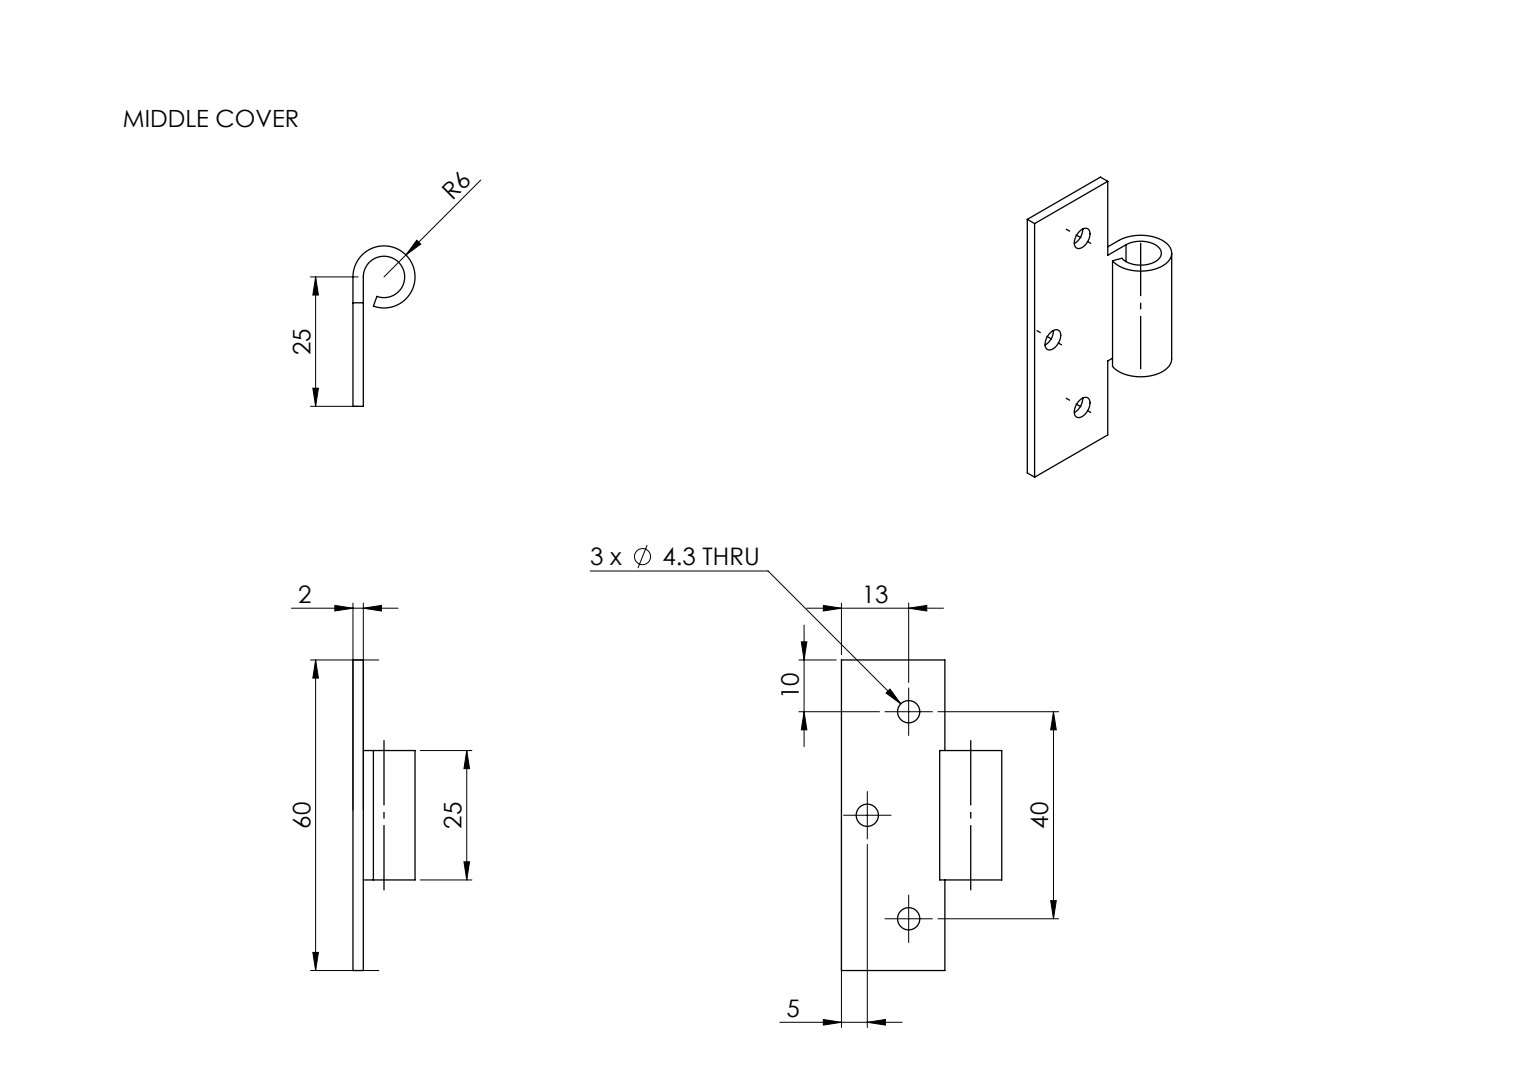
ISO-10303-21;
HEADER;
FILE_DESCRIPTION (('STEP AP214'),
    '1' );
FILE_NAME ('middle cover.step',
    '2026-10-03T20:08:58',
    ( '' ),
    ( '' ),
    'SwSTEP 2.0',
    'SolidWorks 2026',
    '' );
FILE_SCHEMA (( 'AUTOMOTIVE_DESIGN' ));
ENDSEC;

DATA;
#53=ORIENTED_EDGE ( 'NONE', *, *, #9830, .F. ) ;
#58=ORIENTED_EDGE ( 'NONE', *, *, #11138, .F. ) ;
#71=SHAPE_REPRESENTATION ( 'middle cover', ( #12422 ), #3113 ) ;
#124=VECTOR ( 'NONE', #5391, 1000.000000000000000 ) ;
#153=CYLINDRICAL_SURFACE ( 'NONE', #2365, 2.149999999999999023 ) ;
#185=CARTESIAN_POINT ( 'NONE',  ( 15.00000000000003375, -12.49999999999999645, 3.994800001834461867E-31 ) ) ;
#198=DIRECTION ( 'NONE',  ( 1.000000000000000000, 1.849040895279789448E-31, -6.938893903907224680E-17 ) ) ;
#203=CARTESIAN_POINT ( 'NONE',  ( 15.00000000000003375, 30.00000000000001776, -9.742497179615118866E-31 ) ) ;
#207=ORIENTED_EDGE ( 'NONE', *, *, #11487, .T. ) ;
#225=CYLINDRICAL_SURFACE ( 'NONE', #8627, 4.000000000000008882 ) ;
#265=AXIS2_PLACEMENT_3D ( 'NONE', #2707, #625, #8413 ) ;
#298=ORIENTED_EDGE ( 'NONE', *, *, #6646, .F. ) ;
#306=EDGE_CURVE ( 'NONE', #7136, #2489, #7613, .T. ) ;
#307=FACE_OUTER_BOUND ( 'NONE', #3872, .T. ) ;
#324=FACE_BOUND ( 'NONE', #7382, .T. ) ;
#328=DIRECTION ( 'NONE',  ( 1.000000000000000000, 1.849040895279789448E-31, -6.938893903907224680E-17 ) ) ;
#331=CARTESIAN_POINT ( 'NONE',  ( 15.00000000000003375, 12.50000000000000000, -4.062508476441825628E-31 ) ) ;
#347=FACE_OUTER_BOUND ( 'NONE', #4727, .T. ) ;
#349=VERTEX_POINT ( 'NONE', #907 ) ;
#361=LINE ( 'NONE', #555, #3321 ) ;
#392=CARTESIAN_POINT ( 'NONE',  ( 11.00000000000003730, -19.99999999999999645, 12.00000000000003553 ) ) ;
#398=VECTOR ( 'NONE', #6706, 1000.000000000000000 ) ;
#415=ADVANCED_FACE ( 'NONE', ( #12584 ), #4715, .F. ) ;
#499=VERTEX_POINT ( 'NONE', #4254 ) ;
#502=VECTOR ( 'NONE', #1677, 1000.000000000000000 ) ;
#508=LINE ( 'NONE', #572, #8236 ) ;
#527=EDGE_CURVE ( 'NONE', #837, #2437, #10330, .T. ) ;
#534=CARTESIAN_POINT ( 'NONE',  ( 11.00000000000003020, 30.00000000000000000, 25.00000000000007105 ) ) ;
#539=ADVANCED_FACE ( 'NONE', ( #7031 ), #4318, .F. ) ;
#550=AXIS2_PLACEMENT_3D ( 'NONE', #4921, #8783, #1827 ) ;
#555=CARTESIAN_POINT ( 'NONE',  ( 11.00000000000003020, -30.00000000000000000, 25.00000000000007105 ) ) ;
#572=CARTESIAN_POINT ( 'NONE',  ( 11.00000000000003020, 30.00000000000000000, 5.000000000000004441 ) ) ;
#576=EDGE_CURVE ( 'NONE', #499, #3763, #3136, .T. ) ;
#604=ORIENTED_EDGE ( 'NONE', *, *, #7620, .T. ) ;
#619=PLANE ( 'NONE',  #7619 ) ;
#625=DIRECTION ( 'NONE',  ( -1.848892746611746419E-31, -1.000000000000000000, 3.250006781153460502E-32 ) ) ;
#673=CARTESIAN_POINT ( 'NONE',  ( 11.00000000000003020, 30.00000000000000000, 25.00000000000007105 ) ) ;
#705=CARTESIAN_POINT ( 'NONE',  ( 13.63191942669736889, 12.50000000000000000, 3.758770483143645702 ) ) ;
#730=ORIENTED_EDGE ( 'NONE', *, *, #7700, .F. ) ;
#737=DIRECTION ( 'NONE',  ( -1.848892746611746419E-31, -1.000000000000000000, 3.250006781153460502E-32 ) ) ;
#772=EDGE_CURVE ( 'NONE', #5440, #1077, #5854, .T. ) ;
#773=ORIENTED_EDGE ( 'NONE', *, *, #7954, .F. ) ;
#786=UNCERTAINTY_MEASURE_WITH_UNIT (LENGTH_MEASURE( 1.000000000000000082E-05 ), #10711, 'distance_accuracy_value', 'NONE');
#837=VERTEX_POINT ( 'NONE', #4643 ) ;
#845=AXIS2_PLACEMENT_3D ( 'NONE', #4474, #8392, #8331 ) ;
#854=EDGE_CURVE ( 'NONE', #1393, #11974, #1403, .T. ) ;
#855=AXIS2_PLACEMENT_3D ( 'NONE', #331, #8316, #6321 ) ;
#861=DIRECTION ( 'NONE',  ( 1.000000000000000000, 1.849040895279789448E-31, -6.938893903907224680E-17 ) ) ;
#870=SURFACE_STYLE_USAGE ( .BOTH. , #3124 ) ;
#873=AXIS2_PLACEMENT_3D ( 'NONE', #3980, #951, #2044 ) ;
#875=EDGE_LOOP ( 'NONE', ( #207, #9419, #4311, #1916, #9816, #12149, #7760, #7885, #10727, #12727 ) ) ;
#878=LINE ( 'NONE', #9620, #1011 ) ;
#881=DIRECTION ( 'NONE',  ( 1.000000000000000000, 1.848892746611742259E-31, -1.154721252774410375E-34 ) ) ;
#889=ORIENTED_EDGE ( 'NONE', *, *, #10751, .F. ) ;
#902=EDGE_LOOP ( 'NONE', ( #5113, #5119, #7738, #9992 ) ) ;
#907=CARTESIAN_POINT ( 'NONE',  ( 11.00000000000003375, 12.50000000000000000, -7.673627122167892852E-31 ) ) ;
#911=DIRECTION ( 'NONE',  ( 1.000000000000000000, 1.849040895279789448E-31, -6.938893903907224680E-17 ) ) ;
#912=CIRCLE ( 'NONE', #1325, 2.149999999999994138 ) ;
#937=VERTEX_POINT ( 'NONE', #12282 ) ;
#951=DIRECTION ( 'NONE',  ( -1.848892746611746419E-31, -1.000000000000000000, 3.250006781153460502E-32 ) ) ;
#996=ADVANCED_FACE ( 'NONE', ( #11245 ), #1320, .T. ) ;
#1011=VECTOR ( 'NONE', #11836, 1000.000000000000000 ) ;
#1026=ORIENTED_EDGE ( 'NONE', *, *, #306, .F. ) ;
#1038=DIRECTION ( 'NONE',  ( 0.000000000000000000, 0.000000000000000000, -1.000000000000000000 ) ) ;
#1045=VERTEX_POINT ( 'NONE', #5196 ) ;
#1077=VERTEX_POINT ( 'NONE', #673 ) ;
#1088=DIRECTION ( 'NONE',  ( 1.848892746611746419E-31, 1.000000000000000000, -3.250006781153460502E-32 ) ) ;
#1093=CARTESIAN_POINT ( 'NONE',  ( 15.00000000000003375, -12.49999999999999645, 3.994800001834461867E-31 ) ) ;
#1094=DIRECTION ( 'NONE',  ( 1.848892746611746419E-31, 1.000000000000000000, -3.250006781153460502E-32 ) ) ;
#1097=LINE ( 'NONE', #6364, #1940 ) ;
#1099=CARTESIAN_POINT ( 'NONE',  ( 11.00000000000001599, 19.99999999999999645, 12.00000000000003020 ) ) ;
#1105=EDGE_LOOP ( 'NONE', ( #9618, #8342, #10391, #889 ) ) ;
#1109=DIRECTION ( 'NONE',  ( 0.000000000000000000, 0.000000000000000000, -1.000000000000000000 ) ) ;
#1119=ORIENTED_EDGE ( 'NONE', *, *, #12538, .F. ) ;
#1126=CIRCLE ( 'NONE', #4005, 2.149999999999999023 ) ;
#1171=FILL_AREA_STYLE ('',( #3782 ) ) ;
#1172=EDGE_LOOP ( 'NONE', ( #10214, #1741, #1308, #6409 ) ) ;
#1209=ADVANCED_FACE ( 'NONE', ( #7694 ), #6611, .T. ) ;
#1223=CARTESIAN_POINT ( 'NONE',  ( 11.00000000000003020, 30.00000000000000000, 5.000000000000004441 ) ) ;
#1224=EDGE_CURVE ( 'NONE', #5846, #3671, #9624, .T. ) ;
#1232=CARTESIAN_POINT ( 'NONE',  ( 11.00000000000001599, -12.49999999999999645, 3.994800001834461867E-31 ) ) ;
#1233=( NAMED_UNIT ( * ) PLANE_ANGLE_UNIT ( ) SI_UNIT ( $, .RADIAN. ) );
#1240=CARTESIAN_POINT ( 'NONE',  ( 15.00000000000003375, 30.00000000000001776, -4.000000000000008882 ) ) ;
#1250=ORIENTED_EDGE ( 'NONE', *, *, #9318, .T. ) ;
#1294=DIRECTION ( 'NONE',  ( -1.000000000000000000, -1.848892746611742259E-31, 1.154721252774410589E-34 ) ) ;
#1308=ORIENTED_EDGE ( 'NONE', *, *, #6615, .T. ) ;
#1320=PLANE ( 'NONE',  #6991 ) ;
#1325=AXIS2_PLACEMENT_3D ( 'NONE', #1099, #911, #1880 ) ;
#1393=VERTEX_POINT ( 'NONE', #12553 ) ;
#1395=ORIENTED_EDGE ( 'NONE', *, *, #11820, .T. ) ;
#1403=CIRCLE ( 'NONE', #10259, 6.000000000000013323 ) ;
#1417=CIRCLE ( 'NONE', #8620, 4.000000000000008882 ) ;
#1421=DIRECTION ( 'NONE',  ( -1.000000000000000000, -1.848892746611742259E-31, 1.154721252774410589E-34 ) ) ;
#1463=VERTEX_POINT ( 'NONE', #7578 ) ;
#1503=CARTESIAN_POINT ( 'NONE',  ( 11.00000000000003375, -6.123233995736749519E-16, 20.00000000000003553 ) ) ;
#1524=VECTOR ( 'NONE', #6266, 1000.000000000000000 ) ;
#1531=DIRECTION ( 'NONE',  ( 1.000000000000000000, 1.849040895279789448E-31, -6.938893903907224680E-17 ) ) ;
#1542=CARTESIAN_POINT ( 'NONE',  ( 9.000000000000031974, 12.50000000000000000, 5.000000000000004441 ) ) ;
#1549=EDGE_LOOP ( 'NONE', ( #9983, #8678 ) ) ;
#1552=LINE ( 'NONE', #8256, #6421 ) ;
#1558=CARTESIAN_POINT ( 'NONE',  ( 9.000000000000031974, 12.50000000000000000, -6.000000000000017764 ) ) ;
#1567=AXIS2_PLACEMENT_3D ( 'NONE', #7065, #2171, #7130 ) ;
#1590=ORIENTED_EDGE ( 'NONE', *, *, #6258, .T. ) ;
#1604=EDGE_LOOP ( 'NONE', ( #1991, #6241, #1590, #2296, #8881, #12609, #6350, #8005 ) ) ;
#1614=CARTESIAN_POINT ( 'NONE',  ( 15.00000000000003375, 12.50000000000000000, -4.062508476441825628E-31 ) ) ;
#1677=DIRECTION ( 'NONE',  ( -1.000000000000000000, -1.848892746611742259E-31, 1.154721252774410589E-34 ) ) ;
#1706=EDGE_CURVE ( 'NONE', #1045, #7990, #1417, .T. ) ;
#1723=ORIENTED_EDGE ( 'NONE', *, *, #5620, .T. ) ;
#1724=VECTOR ( 'NONE', #2011, 1000.000000000000000 ) ;
#1741=ORIENTED_EDGE ( 'NONE', *, *, #7200, .F. ) ;
#1808=LINE ( 'NONE', #10500, #12392 ) ;
#1818=UNCERTAINTY_MEASURE_WITH_UNIT (LENGTH_MEASURE( 1.000000000000000082E-05 ), #8735, 'distance_accuracy_value', 'NONE');
#1827=DIRECTION ( 'NONE',  ( 0.000000000000000000, 4.478906847412192569E-32, -1.000000000000000000 ) ) ;
#1832=SURFACE_SIDE_STYLE ('',( #9673 ) ) ;
#1842=EDGE_CURVE ( 'NONE', #7990, #8864, #4935, .T. ) ;
#1852=CARTESIAN_POINT ( 'NONE',  ( 15.00000000000003375, -29.99999999999998224, 9.742497179615118866E-31 ) ) ;
#1855=ORIENTED_EDGE ( 'NONE', *, *, #1842, .T. ) ;
#1856=ORIENTED_EDGE ( 'NONE', *, *, #4784, .T. ) ;
#1877=AXIS2_PLACEMENT_3D ( 'NONE', #1503, #5243, #8267 ) ;
#1880=DIRECTION ( 'NONE',  ( 0.000000000000000000, 0.000000000000000000, -1.000000000000000000 ) ) ;
#1889=CARTESIAN_POINT ( 'NONE',  ( 9.000000000000031974, -6.123233995736753463E-16, 20.00000000000003553 ) ) ;
#1898=ORIENTED_EDGE ( 'NONE', *, *, #1224, .T. ) ;
#1906=ORIENTED_EDGE ( 'NONE', *, *, #11800, .T. ) ;
#1916=ORIENTED_EDGE ( 'NONE', *, *, #2991, .T. ) ;
#1918=DIRECTION ( 'NONE',  ( -1.848892746611746419E-31, -1.000000000000000000, 3.250006781153460502E-32 ) ) ;
#1937=LINE ( 'NONE', #10885, #2591 ) ;
#1940=VECTOR ( 'NONE', #5035, 1000.000000000000000 ) ;
#1943=PLANE ( 'NONE',  #2694 ) ;
#1945=ADVANCED_FACE ( 'NONE', ( #4026 ), #225, .F. ) ;
#1977=ORIENTED_EDGE ( 'NONE', *, *, #6329, .F. ) ;
#1981=EDGE_LOOP ( 'NONE', ( #7314, #3852, #8670, #1856 ) ) ;
#1991=ORIENTED_EDGE ( 'NONE', *, *, #9650, .F. ) ;
#2011=DIRECTION ( 'NONE',  ( 1.000000000000000000, 1.849040895279789448E-31, -6.938893903907224680E-17 ) ) ;
#2044=DIRECTION ( 'NONE',  ( 0.000000000000000000, 0.000000000000000000, -1.000000000000000000 ) ) ;
#2046=LINE ( 'NONE', #8931, #12274 ) ;
#2133=FACE_BOUND ( 'NONE', #2564, .T. ) ;
#2138=CARTESIAN_POINT ( 'NONE',  ( 11.00000000000003375, -19.99999999999999645, 14.15000000000003411 ) ) ;
#2156=CARTESIAN_POINT ( 'NONE',  ( 11.00000000000003375, -19.99999999999999645, 12.00000000000003553 ) ) ;
#2171=DIRECTION ( 'NONE',  ( -1.848892746611746419E-31, -1.000000000000000000, 3.250006781153460502E-32 ) ) ;
#2186=ORIENTED_EDGE ( 'NONE', *, *, #9830, .T. ) ;
#2196=FACE_OUTER_BOUND ( 'NONE', #11712, .T. ) ;
#2212=VECTOR ( 'NONE', #3263, 1000.000000000000000 ) ;
#2247=EDGE_CURVE ( 'NONE', #2437, #7453, #7218, .T. ) ;
#2257=VECTOR ( 'NONE', #11038, 1000.000000000000000 ) ;
#2279=CARTESIAN_POINT ( 'NONE',  ( 12.94787914004602847, -12.49999999999999645, 5.638155724715463890 ) ) ;
#2296=ORIENTED_EDGE ( 'NONE', *, *, #10876, .F. ) ;
#2300=DIRECTION ( 'NONE',  ( 0.000000000000000000, 0.000000000000000000, -1.000000000000000000 ) ) ;
#2315=CARTESIAN_POINT ( 'NONE',  ( 15.00000000000003375, 30.00000000000001776, -9.742497179615118866E-31 ) ) ;
#2321=CARTESIAN_POINT ( 'NONE',  ( 11.00000000000003375, -6.123233995736745575E-16, 20.00000000000003553 ) ) ;
#2341=DIRECTION ( 'NONE',  ( 0.3420201433256680468, 7.946868433027814422E-32, -0.9396926207859086499 ) ) ;
#2353=LINE ( 'NONE', #10308, #1524 ) ;
#2354=ADVANCED_FACE ( 'NONE', ( #324, #10031, #2133, #8247 ), #8180, .T. ) ;
#2365=AXIS2_PLACEMENT_3D ( 'NONE', #2156, #6804, #3958 ) ;
#2389=FACE_OUTER_BOUND ( 'NONE', #5721, .T. ) ;
#2390=EDGE_LOOP ( 'NONE', ( #9885, #4090, #6511, #7356 ) ) ;
#2418=LINE ( 'NONE', #7178, #11409 ) ;
#2429=DIRECTION ( 'NONE',  ( -0.3420201433256680468, -7.946868433027813328E-32, 0.9396926207859086499 ) ) ;
#2437=VERTEX_POINT ( 'NONE', #12311 ) ;
#2447=FACE_OUTER_BOUND ( 'NONE', #1981, .T. ) ;
#2466=EDGE_LOOP ( 'NONE', ( #12293, #4442 ) ) ;
#2468=CARTESIAN_POINT ( 'NONE',  ( 21.00000000000003197, -30.00000000000000000, 5.000000000000011546 ) ) ;
#2489=VERTEX_POINT ( 'NONE', #1542 ) ;
#2522=CIRCLE ( 'NONE', #855, 4.000000000000008882 ) ;
#2533=ORIENTED_EDGE ( 'NONE', *, *, #6615, .F. ) ;
#2564=EDGE_LOOP ( 'NONE', ( #58, #5215 ) ) ;
#2591=VECTOR ( 'NONE', #6970, 1000.000000000000000 ) ;
#2614=ORIENTED_EDGE ( 'NONE', *, *, #1706, .F. ) ;
#2636=ORIENTED_EDGE ( 'NONE', *, *, #11706, .F. ) ;
#2663=CARTESIAN_POINT ( 'NONE',  ( 9.000000000000017764, 19.99999999999999645, 14.15000000000002345 ) ) ;
#2688=ORIENTED_EDGE ( 'NONE', *, *, #7898, .T. ) ;
#2694=AXIS2_PLACEMENT_3D ( 'NONE', #203, #4132, #11745 ) ;
#2703=ORIENTED_EDGE ( 'NONE', *, *, #6258, .F. ) ;
#2707=CARTESIAN_POINT ( 'NONE',  ( 15.00000000000003375, 12.50000000000000000, -4.062508476441825628E-31 ) ) ;
#2709=PRODUCT ( 'middle cover', 'middle cover', '', ( #4085 ) ) ;
#2746=CLOSED_SHELL ( 'NONE', ( #9617, #539, #4850, #4582, #5554, #3059, #5777, #10912, #10366, #6759, #10943, #2354, #1945, #996, #1209, #7851, #11352, #7779, #415, #8563, #6522, #11560 ) ) ;
#2791=CARTESIAN_POINT ( 'NONE',  ( 15.00000000000003375, 12.50000000000000000, -4.062508476441825628E-31 ) ) ;
#2821=DIRECTION ( 'NONE',  ( 0.000000000000000000, 0.000000000000000000, -1.000000000000000000 ) ) ;
#2833=SURFACE_STYLE_FILL_AREA ( #1171 ) ;
#2835=ORIENTED_EDGE ( 'NONE', *, *, #11243, .T. ) ;
#2876=EDGE_LOOP ( 'NONE', ( #4069, #1855, #2636, #1119 ) ) ;
#2890=FILL_AREA_STYLE ('',( #12540 ) ) ;
#2896=( NAMED_UNIT ( * ) SI_UNIT ( $, .STERADIAN. ) SOLID_ANGLE_UNIT ( ) );
#2897=AXIS2_PLACEMENT_3D ( 'NONE', #9255, #5155, #7153 ) ;
#2902=DIRECTION ( 'NONE',  ( -1.848892746611746419E-31, -1.000000000000000000, 3.250006781153460502E-32 ) ) ;
#2991=EDGE_CURVE ( 'NONE', #11641, #9518, #878, .T. ) ;
#3022=DIRECTION ( 'NONE',  ( -1.848892746611746419E-31, -1.000000000000000000, 3.250006781153460502E-32 ) ) ;
#3044=VECTOR ( 'NONE', #5677, 1000.000000000000000 ) ;
#3059=ADVANCED_FACE ( 'NONE', ( #8608 ), #9684, .F. ) ;
#3072=LINE ( 'NONE', #10904, #2257 ) ;
#3076=DIRECTION ( 'NONE',  ( 1.000000000000000000, 1.849040895279789448E-31, -6.938893903907224680E-17 ) ) ;
#3081=CARTESIAN_POINT ( 'NONE',  ( 13.63191942669736889, 30.00000000000001776, 3.758770483143646146 ) ) ;
#3113=( GEOMETRIC_REPRESENTATION_CONTEXT ( 3 ) GLOBAL_UNCERTAINTY_ASSIGNED_CONTEXT ( ( #10448 ) ) GLOBAL_UNIT_ASSIGNED_CONTEXT ( ( #6131, #3843, #12064 ) ) REPRESENTATION_CONTEXT ( 'NONE', 'WORKASPACE' ) );
#3124=SURFACE_SIDE_STYLE ('',( #2833 ) ) ;
#3136=CIRCLE ( 'NONE', #4179, 4.000000000000008882 ) ;
#3156=CARTESIAN_POINT ( 'NONE',  ( 9.000000000000017764, 19.99999999999999645, 12.00000000000003020 ) ) ;
#3169=VERTEX_POINT ( 'NONE', #3337 ) ;
#3176=LINE ( 'NONE', #5517, #3290 ) ;
#3182=CARTESIAN_POINT ( 'NONE',  ( 11.00000000000003375, -6.123233995736745575E-16, 20.00000000000003553 ) ) ;
#3193=ORIENTED_EDGE ( 'NONE', *, *, #3431, .T. ) ;
#3196=AXIS2_PLACEMENT_3D ( 'NONE', #7099, #11084, #5225 ) ;
#3232=DIRECTION ( 'NONE',  ( -1.848892746611746419E-31, -1.000000000000000000, 3.250006781153460502E-32 ) ) ;
#3248=DIRECTION ( 'NONE',  ( 1.848892746611746419E-31, 1.000000000000000000, -3.250006781153460502E-32 ) ) ;
#3251=DIRECTION ( 'NONE',  ( -1.154721252774002618E-34, 1.982541115402070533E-16, 1.000000000000000000 ) ) ;
#3263=DIRECTION ( 'NONE',  ( -1.848892746611746419E-31, -1.000000000000000000, 3.250006781153460502E-32 ) ) ;
#3276=ORIENTED_EDGE ( 'NONE', *, *, #8405, .T. ) ;
#3277=CARTESIAN_POINT ( 'NONE',  ( 15.00000000000003375, 12.50000000000000000, -4.062508476441825628E-31 ) ) ;
#3290=VECTOR ( 'NONE', #8410, 1000.000000000000000 ) ;
#3291=CYLINDRICAL_SURFACE ( 'NONE', #8137, 6.000000000000013323 ) ;
#3298=DIRECTION ( 'NONE',  ( 1.848892746611746419E-31, 1.000000000000000000, -3.250006781153460502E-32 ) ) ;
#3304=CARTESIAN_POINT ( 'NONE',  ( 9.000000000000017764, -12.50000000000000178, 5.000000000000007994 ) ) ;
#3321=VECTOR ( 'NONE', #8467, 1000.000000000000000 ) ;
#3337=CARTESIAN_POINT ( 'NONE',  ( 9.000000000000035527, -19.99999999999999645, 9.850000000000035172 ) ) ;
#3356=VERTEX_POINT ( 'NONE', #10454 ) ;
#3363=PRODUCT_DEFINITION_CONTEXT ( 'detailed design', #10762, 'design' ) ;
#3431=EDGE_CURVE ( 'NONE', #4174, #10853, #4732, .T. ) ;
#3442=CIRCLE ( 'NONE', #550, 2.149999999999992362 ) ;
#3465=DIRECTION ( 'NONE',  ( -1.000000000000000000, -1.848892746611742259E-31, 1.154721252774410589E-34 ) ) ;
#3468=EDGE_LOOP ( 'NONE', ( #12230, #6935, #2835, #7511 ) ) ;
#3482=DIRECTION ( 'NONE',  ( 1.000000000000000000, 1.849040895279789448E-31, -6.938893903907224680E-17 ) ) ;
#3512=AXIS2_PLACEMENT_3D ( 'NONE', #9008, #12247, #7160 ) ;
#3526=CYLINDRICAL_SURFACE ( 'NONE', #5889, 6.000000000000013323 ) ;
#3541=CIRCLE ( 'NONE', #1877, 2.149999999999992362 ) ;
#3551=AXIS2_PLACEMENT_3D ( 'NONE', #10954, #10759, #1038 ) ;
#3562=CARTESIAN_POINT ( 'NONE',  ( 9.000000000000028422, 30.00000000000000000, -9.742497179615118866E-31 ) ) ;
#3595=PLANE ( 'NONE',  #8237 ) ;
#3606=DIRECTION ( 'NONE',  ( -1.000000000000000000, -1.848892746611742259E-31, 1.154721252774410589E-34 ) ) ;
#3671=VERTEX_POINT ( 'NONE', #5108 ) ;
#3692=EDGE_CURVE ( 'NONE', #4808, #7388, #6922, .T. ) ;
#3751=DIRECTION ( 'NONE',  ( 1.000000000000000000, 1.849040895279789448E-31, -6.938893903907224680E-17 ) ) ;
#3753=CIRCLE ( 'NONE', #8677, 6.000000000000013323 ) ;
#3763=VERTEX_POINT ( 'NONE', #11287 ) ;
#3782=FILL_AREA_STYLE_COLOUR ( '', #9870 ) ;
#3808=ORIENTED_EDGE ( 'NONE', *, *, #1842, .F. ) ;
#3809=CIRCLE ( 'NONE', #5452, 2.149999999999999023 ) ;
#3816=CARTESIAN_POINT ( 'NONE',  ( 21.00000000000003197, 12.50000000000000888, 5.000000000000004441 ) ) ;
#3843=( NAMED_UNIT ( * ) PLANE_ANGLE_UNIT ( ) SI_UNIT ( $, .RADIAN. ) );
#3852=ORIENTED_EDGE ( 'NONE', *, *, #6020, .F. ) ;
#3872=EDGE_LOOP ( 'NONE', ( #8759, #6873, #11254, #9704 ) ) ;
#3931=CARTESIAN_POINT ( 'NONE',  ( 15.00000000000003375, -12.49999999999999645, 3.994800001834461867E-31 ) ) ;
#3936=DIRECTION ( 'NONE',  ( 1.000000000000000000, 1.848892746611742259E-31, -1.154721252774410375E-34 ) ) ;
#3941=LINE ( 'NONE', #2138, #7192 ) ;
#3953=DIRECTION ( 'NONE',  ( 0.000000000000000000, 0.000000000000000000, -1.000000000000000000 ) ) ;
#3958=DIRECTION ( 'NONE',  ( 0.000000000000000000, 0.000000000000000000, -1.000000000000000000 ) ) ;
#3980=CARTESIAN_POINT ( 'NONE',  ( 15.00000000000003375, 12.50000000000000000, -4.062508476441825628E-31 ) ) ;
#4005=AXIS2_PLACEMENT_3D ( 'NONE', #3156, #10855, #5072 ) ;
#4018=CARTESIAN_POINT ( 'NONE',  ( 9.000000000000035527, -30.00000000000000000, 25.00000000000007105 ) ) ;
#4026=FACE_OUTER_BOUND ( 'NONE', #1105, .T. ) ;
#4042=ORIENTED_EDGE ( 'NONE', *, *, #11702, .T. ) ;
#4049=EDGE_CURVE ( 'NONE', #4417, #3169, #12232, .T. ) ;
#4063=DIRECTION ( 'NONE',  ( 1.000000000000000000, 1.849040895279789448E-31, -6.938893903907224680E-17 ) ) ;
#4069=ORIENTED_EDGE ( 'NONE', *, *, #6576, .F. ) ;
#4085=PRODUCT_CONTEXT ( 'NONE', #10101, 'mechanical' ) ;
#4090=ORIENTED_EDGE ( 'NONE', *, *, #7954, .T. ) ;
#4091=AXIS2_PLACEMENT_3D ( 'NONE', #392, #9145, #5167 ) ;
#4107=DIRECTION ( 'NONE',  ( 6.938893903907224680E-17, -3.250006781153453386E-32, 1.000000000000000000 ) ) ;
#4132=DIRECTION ( 'NONE',  ( -1.848892746611742259E-31, 1.000000000000000000, -3.250006781153460502E-32 ) ) ;
#4148=VECTOR ( 'NONE', #2341, 1000.000000000000000 ) ;
#4174=VERTEX_POINT ( 'NONE', #9433 ) ;
#4178=DIRECTION ( 'NONE',  ( 1.000000000000000000, 1.849040895279789448E-31, -6.938893903907224680E-17 ) ) ;
#4179=AXIS2_PLACEMENT_3D ( 'NONE', #9968, #1094, #11992 ) ;
#4214=DIRECTION ( 'NONE',  ( 0.000000000000000000, 0.000000000000000000, -1.000000000000000000 ) ) ;
#4236=CARTESIAN_POINT ( 'NONE',  ( 9.000000000000028422, -30.00000000000000000, 1.387778780781457755E-16 ) ) ;
#4254=CARTESIAN_POINT ( 'NONE',  ( 15.00000000000003375, -12.49999999999999645, 4.000000000000000000 ) ) ;
#4311=ORIENTED_EDGE ( 'NONE', *, *, #10751, .T. ) ;
#4318=CYLINDRICAL_SURFACE ( 'NONE', #9682, 2.149999999999999023 ) ;
#4321=FACE_OUTER_BOUND ( 'NONE', #875, .T. ) ;
#4352=FACE_OUTER_BOUND ( 'NONE', #4551, .T. ) ;
#4369=DIRECTION ( 'NONE',  ( 0.000000000000000000, 0.000000000000000000, -1.000000000000000000 ) ) ;
#4401=CARTESIAN_POINT ( 'NONE',  ( 11.00000000000003375, -6.123233995736748533E-16, 17.85000000000004405 ) ) ;
#4417=VERTEX_POINT ( 'NONE', #4944 ) ;
#4442=ORIENTED_EDGE ( 'NONE', *, *, #4049, .T. ) ;
#4474=CARTESIAN_POINT ( 'NONE',  ( 11.00000000000002665, 12.50000000000000000, -6.000000000000017764 ) ) ;
#4491=CARTESIAN_POINT ( 'NONE',  ( 11.00000000000003020, 30.00000000000000000, 25.00000000000007105 ) ) ;
#4504=DIRECTION ( 'NONE',  ( -1.848892746611746419E-31, -1.000000000000000000, 3.250006781153460502E-32 ) ) ;
#4551=EDGE_LOOP ( 'NONE', ( #1395, #8552, #11834, #1977 ) ) ;
#4582=ADVANCED_FACE ( 'NONE', ( #4352 ), #3526, .T. ) ;
#4643=CARTESIAN_POINT ( 'NONE',  ( 15.00000000000003375, -12.49999999999999645, 6.000000000000000000 ) ) ;
#4648=ORIENTED_EDGE ( 'NONE', *, *, #1706, .T. ) ;
#4659=CARTESIAN_POINT ( 'NONE',  ( 13.63191942669736889, -12.49999999999999645, 3.758770483143645702 ) ) ;
#4669=LINE ( 'NONE', #5573, #9988 ) ;
#4715=PLANE ( 'NONE',  #9708 ) ;
#4727=EDGE_LOOP ( 'NONE', ( #10466, #12619, #12733, #11650, #7834, #9442, #1723, #4042, #7966, #4648 ) ) ;
#4732=LINE ( 'NONE', #8659, #9928 ) ;
#4760=EDGE_CURVE ( 'NONE', #1393, #837, #12604, .T. ) ;
#4784=EDGE_CURVE ( 'NONE', #7388, #10795, #3442, .T. ) ;
#4794=AXIS2_PLACEMENT_3D ( 'NONE', #11149, #3248, #9009 ) ;
#4808=VERTEX_POINT ( 'NONE', #11569 ) ;
#4850=ADVANCED_FACE ( 'NONE', ( #4857 ), #5757, .F. ) ;
#4857=FACE_OUTER_BOUND ( 'NONE', #5580, .T. ) ;
#4859=DIRECTION ( 'NONE',  ( 0.000000000000000000, 0.000000000000000000, -1.000000000000000000 ) ) ;
#4921=CARTESIAN_POINT ( 'NONE',  ( 11.00000000000003375, -6.123233995736749519E-16, 20.00000000000003553 ) ) ;
#4928=EDGE_LOOP ( 'NONE', ( #12326, #2688 ) ) ;
#4935=LINE ( 'NONE', #3081, #12145 ) ;
#4944=CARTESIAN_POINT ( 'NONE',  ( 9.000000000000035527, -19.99999999999999645, 14.15000000000002878 ) ) ;
#4959=MECHANICAL_DESIGN_GEOMETRIC_PRESENTATION_REPRESENTATION('',(#12372),#10279);
#4978=ORIENTED_EDGE ( 'NONE', *, *, #6766, .T. ) ;
#4980=EDGE_CURVE ( 'NONE', #349, #11641, #6137, .T. ) ;
#4984=EDGE_CURVE ( 'NONE', #9732, #3763, #4985, .T. ) ;
#4985=LINE ( 'NONE', #1240, #10200 ) ;
#5000=ORIENTED_EDGE ( 'NONE', *, *, #5663, .T. ) ;
#5027=DIRECTION ( 'NONE',  ( 0.000000000000000000, 0.000000000000000000, 1.000000000000000000 ) ) ;
#5035=DIRECTION ( 'NONE',  ( -0.3420201433256680468, -7.946868433027814422E-32, 0.9396926207859086499 ) ) ;
#5064=DIRECTION ( 'NONE',  ( 0.000000000000000000, 0.000000000000000000, -1.000000000000000000 ) ) ;
#5072=DIRECTION ( 'NONE',  ( 0.000000000000000000, 0.000000000000000000, -1.000000000000000000 ) ) ;
#5108=CARTESIAN_POINT ( 'NONE',  ( 11.00000000000001599, 19.99999999999999645, 14.15000000000001812 ) ) ;
#5113=ORIENTED_EDGE ( 'NONE', *, *, #8405, .F. ) ;
#5119=ORIENTED_EDGE ( 'NONE', *, *, #12552, .F. ) ;
#5139=EDGE_LOOP ( 'NONE', ( #8872, #9117, #2186, #8240 ) ) ;
#5155=DIRECTION ( 'NONE',  ( 1.000000000000000000, 1.849040895279789448E-31, -6.938893903907224680E-17 ) ) ;
#5167=DIRECTION ( 'NONE',  ( 0.000000000000000000, 0.000000000000000000, -1.000000000000000000 ) ) ;
#5170=SHAPE_REPRESENTATION_RELATIONSHIP ( 'NONE' , 'NONE' ,  #71, #11261 ) ;
#5177=DIRECTION ( 'NONE',  ( -1.848892746611746419E-31, -1.000000000000000000, 3.250006781153460502E-32 ) ) ;
#5196=CARTESIAN_POINT ( 'NONE',  ( 15.00000000000003375, 12.50000000000000000, 4.000000000000000000 ) ) ;
#5215=ORIENTED_EDGE ( 'NONE', *, *, #9098, .F. ) ;
#5225=DIRECTION ( 'NONE',  ( -1.154721252774410375E-34, -3.250006781153453386E-32, 1.000000000000000000 ) ) ;
#5243=DIRECTION ( 'NONE',  ( 1.000000000000000000, 1.849040895279789448E-31, -6.938893903907224680E-17 ) ) ;
#5269=CARTESIAN_POINT ( 'NONE',  ( 9.000000000000035527, -19.99999999999999645, 12.00000000000003553 ) ) ;
#5309=VERTEX_POINT ( 'NONE', #11932 ) ;
#5339=CYLINDRICAL_SURFACE ( 'NONE', #2897, 2.149999999999999023 ) ;
#5376=CYLINDRICAL_SURFACE ( 'NONE', #1567, 4.000000000000008882 ) ;
#5391=DIRECTION ( 'NONE',  ( -1.848892746611746419E-31, -1.000000000000000000, 3.250006781153460502E-32 ) ) ;
#5440=VERTEX_POINT ( 'NONE', #1223 ) ;
#5446=ORIENTED_EDGE ( 'NONE', *, *, #1224, .F. ) ;
#5447=EDGE_CURVE ( 'NONE', #10646, #3356, #12707, .T. ) ;
#5452=AXIS2_PLACEMENT_3D ( 'NONE', #11950, #11756, #4859 ) ;
#5454=DIRECTION ( 'NONE',  ( -6.938893903907224680E-17, 3.250006781153453386E-32, -1.000000000000000000 ) ) ;
#5473=ORIENTED_EDGE ( 'NONE', *, *, #6786, .F. ) ;
#5493=DIRECTION ( 'NONE',  ( 6.938893903907224680E-17, -3.250006781153453386E-32, 1.000000000000000000 ) ) ;
#5517=CARTESIAN_POINT ( 'NONE',  ( 11.00000000000003020, -30.00000000000000000, 9.757543507305644146E-31 ) ) ;
#5528=LINE ( 'NONE', #12430, #9538 ) ;
#5530=LINE ( 'NONE', #10411, #6701 ) ;
#5554=ADVANCED_FACE ( 'NONE', ( #307 ), #3291, .T. ) ;
#5572=EDGE_CURVE ( 'NONE', #4174, #8613, #11907, .T. ) ;
#5573=CARTESIAN_POINT ( 'NONE',  ( 11.00000000000003020, 30.00000000000000000, 25.00000000000007105 ) ) ;
#5580=EDGE_LOOP ( 'NONE', ( #9288, #9188, #10138, #2533 ) ) ;
#5582=ORIENTED_EDGE ( 'NONE', *, *, #11243, .F. ) ;
#5597=AXIS2_PLACEMENT_3D ( 'NONE', #5749, #6791, #10511 ) ;
#5618=CARTESIAN_POINT ( 'NONE',  ( 11.00000000000003730, -19.99999999999999645, 14.15000000000002345 ) ) ;
#5620=EDGE_CURVE ( 'NONE', #937, #349, #2046, .T. ) ;
#5627=ORIENTED_EDGE ( 'NONE', *, *, #11487, .F. ) ;
#5650=LINE ( 'NONE', #9434, #5853 ) ;
#5663=EDGE_CURVE ( 'NONE', #7136, #7453, #11453, .T. ) ;
#5677=DIRECTION ( 'NONE',  ( -1.848892746611746419E-31, -1.000000000000000000, 3.250006781153460502E-32 ) ) ;
#5707=CARTESIAN_POINT ( 'NONE',  ( 0.000000000000000000, 0.000000000000000000, 0.000000000000000000 ) ) ;
#5721=EDGE_LOOP ( 'NONE', ( #7456, #4978, #7459, #9414 ) ) ;
#5735=DIRECTION ( 'NONE',  ( -1.848892746611746419E-31, -1.000000000000000000, 3.250006781153460502E-32 ) ) ;
#5749=CARTESIAN_POINT ( 'NONE',  ( 15.00000000000003375, -12.49999999999999645, 3.994800001834461867E-31 ) ) ;
#5757=CYLINDRICAL_SURFACE ( 'NONE', #6302, 2.149999999999999023 ) ;
#5777=ADVANCED_FACE ( 'NONE', ( #10252 ), #5376, .F. ) ;
#5817=DIRECTION ( 'NONE',  ( 0.000000000000000000, 4.478906847412178337E-32, -1.000000000000000000 ) ) ;
#5832=EDGE_CURVE ( 'NONE', #1077, #10196, #4669, .T. ) ;
#5846=VERTEX_POINT ( 'NONE', #11307 ) ;
#5853=VECTOR ( 'NONE', #3606, 1000.000000000000000 ) ;
#5854=LINE ( 'NONE', #8624, #398 ) ;
#5889=AXIS2_PLACEMENT_3D ( 'NONE', #7381, #12350, #9413 ) ;
#5931=CARTESIAN_POINT ( 'NONE',  ( 15.00000000000003375, 12.50000000000000000, -6.000000000000000000 ) ) ;
#5935=AXIS2_PLACEMENT_3D ( 'NONE', #3931, #1088, #5027 ) ;
#5985=CARTESIAN_POINT ( 'NONE',  ( 11.00000000000003375, -3.490243377569943242E-16, 22.15000000000002345 ) ) ;
#5992=DIRECTION ( 'NONE',  ( 0.000000000000000000, 4.478906847412178337E-32, -1.000000000000000000 ) ) ;
#6012=FACE_OUTER_BOUND ( 'NONE', #1172, .T. ) ;
#6016=CARTESIAN_POINT ( 'NONE',  ( 11.00000000000003730, -19.99999999999999645, 12.00000000000003553 ) ) ;
#6020=EDGE_CURVE ( 'NONE', #4808, #5309, #9787, .T. ) ;
#6056=DIRECTION ( 'NONE',  ( 0.000000000000000000, 4.478906847412178337E-32, -1.000000000000000000 ) ) ;
#6060=AXIS2_PLACEMENT_3D ( 'NONE', #185, #3298, #7972 ) ;
#6079=ORIENTED_EDGE ( 'NONE', *, *, #11724, .T. ) ;
#6127=DIRECTION ( 'NONE',  ( -1.848892746611746419E-31, -1.000000000000000000, 1.982541115402070533E-16 ) ) ;
#6131=( LENGTH_UNIT ( ) NAMED_UNIT ( * ) SI_UNIT ( .MILLI., .METRE. ) );
#6137=LINE ( 'NONE', #12072, #2212 ) ;
#6227=CIRCLE ( 'NONE', #873, 4.000000000000008882 ) ;
#6241=ORIENTED_EDGE ( 'NONE', *, *, #772, .T. ) ;
#6258=EDGE_CURVE ( 'NONE', #1077, #12174, #8387, .T. ) ;
#6266=DIRECTION ( 'NONE',  ( 1.000000000000000000, 1.849040895279789448E-31, -6.938893903907224680E-17 ) ) ;
#6302=AXIS2_PLACEMENT_3D ( 'NONE', #10585, #861, #3953 ) ;
#6321=DIRECTION ( 'NONE',  ( 0.000000000000000000, 0.000000000000000000, -1.000000000000000000 ) ) ;
#6329=EDGE_CURVE ( 'NONE', #8944, #2437, #11738, .T. ) ;
#6341=DIRECTION ( 'NONE',  ( -0.9396926207859086499, -1.281224895503606024E-31, -0.3420201433256680468 ) ) ;
#6350=ORIENTED_EDGE ( 'NONE', *, *, #4980, .F. ) ;
#6364=CARTESIAN_POINT ( 'NONE',  ( 12.94787914004603557, 12.50000000000000000, 5.638155724715463890 ) ) ;
#6401=CARTESIAN_POINT ( 'NONE',  ( 9.000000000000035527, 30.00000000000000000, 25.00000000000007105 ) ) ;
#6409=ORIENTED_EDGE ( 'NONE', *, *, #11138, .T. ) ;
#6421=VECTOR ( 'NONE', #1421, 1000.000000000000000 ) ;
#6428=DIRECTION ( 'NONE',  ( 1.000000000000000000, 0.000000000000000000, 0.000000000000000000 ) ) ;
#6484=CARTESIAN_POINT ( 'NONE',  ( 9.000000000000031974, 12.50000000000000000, -1.576761677324514786E-16 ) ) ;
#6491=FACE_BOUND ( 'NONE', #4928, .T. ) ;
#6511=ORIENTED_EDGE ( 'NONE', *, *, #11924, .T. ) ;
#6517=LINE ( 'NONE', #6648, #10888 ) ;
#6522=ADVANCED_FACE ( 'NONE', ( #2447 ), #10209, .F. ) ;
#6554=EDGE_LOOP ( 'NONE', ( #2614, #3276, #5627, #3808 ) ) ;
#6556=CARTESIAN_POINT ( 'NONE',  ( 9.000000000000028422, 30.00000000000000000, -5.960102014102692796E-16 ) ) ;
#6576=EDGE_CURVE ( 'NONE', #7990, #11974, #1097, .T. ) ;
#6589=CIRCLE ( 'NONE', #5935, 4.000000000000008882 ) ;
#6611=CYLINDRICAL_SURFACE ( 'NONE', #12329, 6.000000000000013323 ) ;
#6615=EDGE_CURVE ( 'NONE', #3169, #1463, #7401, .T. ) ;
#6618=( NAMED_UNIT ( * ) PLANE_ANGLE_UNIT ( ) SI_UNIT ( $, .RADIAN. ) );
#6644=DIRECTION ( 'NONE',  ( 0.000000000000000000, 0.000000000000000000, -1.000000000000000000 ) ) ;
#6646=EDGE_CURVE ( 'NONE', #9518, #10853, #5650, .T. ) ;
#6648=CARTESIAN_POINT ( 'NONE',  ( 9.000000000000035527, 30.00000000000000000, 25.00000000000007105 ) ) ;
#6652=LINE ( 'NONE', #3562, #10309 ) ;
#6678=AXIS2_PLACEMENT_3D ( 'NONE', #5269, #4178, #4369 ) ;
#6679=CARTESIAN_POINT ( 'NONE',  ( 11.00000000000003020, -30.00000000000000000, 5.000000000000011546 ) ) ;
#6701=VECTOR ( 'NONE', #4504, 1000.000000000000000 ) ;
#6706=DIRECTION ( 'NONE',  ( 6.938893903907224680E-17, -3.250006781153453386E-32, 1.000000000000000000 ) ) ;
#6713=DIRECTION ( 'NONE',  ( -1.154721252774410589E-34, -3.250006781153453386E-32, 1.000000000000000000 ) ) ;
#6730=DIRECTION ( 'NONE',  ( 1.725633230170963324E-31, 1.000000000000000000, -1.982541115402070533E-16 ) ) ;
#6739=SURFACE_STYLE_USAGE ( .BOTH. , #1832 ) ;
#6752=FACE_OUTER_BOUND ( 'NONE', #5139, .T. ) ;
#6759=ADVANCED_FACE ( 'NONE', ( #6752 ), #10661, .F. ) ;
#6766=EDGE_CURVE ( 'NONE', #10646, #3671, #5528, .T. ) ;
#6786=EDGE_CURVE ( 'NONE', #3356, #10646, #1126, .T. ) ;
#6791=DIRECTION ( 'NONE',  ( 1.848892746611746419E-31, 1.000000000000000000, -3.250006781153460502E-32 ) ) ;
#6804=DIRECTION ( 'NONE',  ( 1.000000000000000000, 1.849040895279789448E-31, -6.938893903907224680E-17 ) ) ;
#6826=CARTESIAN_POINT ( 'NONE',  ( 12.94787914004603202, 30.00000000000000000, 5.638155724715463890 ) ) ;
#6873=ORIENTED_EDGE ( 'NONE', *, *, #6329, .T. ) ;
#6889=LINE ( 'NONE', #6826, #8892 ) ;
#6898=PRODUCT_DEFINITION ( 'UNKNOWN', '', #6946, #3363 ) ;
#6922=LINE ( 'NONE', #10829, #1724 ) ;
#6925=CARTESIAN_POINT ( 'NONE',  ( 15.00000000000003375, 30.00000000000001776, 6.000000000000013323 ) ) ;
#6935=ORIENTED_EDGE ( 'NONE', *, *, #8711, .T. ) ;
#6946=PRODUCT_DEFINITION_FORMATION_WITH_SPECIFIED_SOURCE ( 'ANY', '', #2709, .NOT_KNOWN. ) ;
#6970=DIRECTION ( 'NONE',  ( -1.725633230170963324E-31, -1.000000000000000000, 1.982541115402070533E-16 ) ) ;
#6991=AXIS2_PLACEMENT_3D ( 'NONE', #7380, #6341, #2429 ) ;
#7031=FACE_OUTER_BOUND ( 'NONE', #3468, .T. ) ;
#7041=PRESENTATION_STYLE_ASSIGNMENT (( #870 ) ) ;
#7065=CARTESIAN_POINT ( 'NONE',  ( 15.00000000000003375, 30.00000000000001776, -9.742497179615118866E-31 ) ) ;
#7066=DIRECTION ( 'NONE',  ( -1.848892746611746419E-31, -1.000000000000000000, 3.250006781153460502E-32 ) ) ;
#7070=EDGE_LOOP ( 'NONE', ( #53, #2703, #12286, #1250 ) ) ;
#7099=CARTESIAN_POINT ( 'NONE',  ( 11.00000000000001243, -12.50000000000000000, -6.000000000000017764 ) ) ;
#7130=DIRECTION ( 'NONE',  ( 0.000000000000000000, 0.000000000000000000, -1.000000000000000000 ) ) ;
#7135=EDGE_LOOP ( 'NONE', ( #11504, #8472, #11979, #773 ) ) ;
#7136=VERTEX_POINT ( 'NONE', #6484 ) ;
#7138=ORIENTED_EDGE ( 'NONE', *, *, #9318, .F. ) ;
#7153=DIRECTION ( 'NONE',  ( 0.000000000000000000, 0.000000000000000000, -1.000000000000000000 ) ) ;
#7160=DIRECTION ( 'NONE',  ( -6.938893903907224680E-17, 3.250006781153453386E-32, -1.000000000000000000 ) ) ;
#7178=CARTESIAN_POINT ( 'NONE',  ( 9.000000000000017764, -12.49999999999999112, -6.000000000000038192 ) ) ;
#7190=DIRECTION ( 'NONE',  ( -1.848892746611746419E-31, -1.000000000000000000, 3.250006781153460502E-32 ) ) ;
#7192=VECTOR ( 'NONE', #4063, 1000.000000000000000 ) ;
#7200=EDGE_CURVE ( 'NONE', #3169, #4417, #3809, .T. ) ;
#7218=CIRCLE ( 'NONE', #9253, 6.000000000000013323 ) ;
#7239=CIRCLE ( 'NONE', #5597, 4.000000000000008882 ) ;
#7314=ORIENTED_EDGE ( 'NONE', *, *, #8711, .F. ) ;
#7335=VECTOR ( 'NONE', #4107, 1000.000000000000000 ) ;
#7356=ORIENTED_EDGE ( 'NONE', *, *, #5832, .F. ) ;
#7380=CARTESIAN_POINT ( 'NONE',  ( 12.94787914004603202, 30.00000000000000000, 5.638155724715463890 ) ) ;
#7381=CARTESIAN_POINT ( 'NONE',  ( 15.00000000000003375, 30.00000000000001776, -9.742497179615118866E-31 ) ) ;
#7382=EDGE_LOOP ( 'NONE', ( #5446, #730 ) ) ;
#7388=VERTEX_POINT ( 'NONE', #4401 ) ;
#7392=DIRECTION ( 'NONE',  ( 0.000000000000000000, 0.000000000000000000, 1.000000000000000000 ) ) ;
#7399=ORIENTED_EDGE ( 'NONE', *, *, #8671, .F. ) ;
#7401=LINE ( 'NONE', #11332, #7499 ) ;
#7453=VERTEX_POINT ( 'NONE', #10235 ) ;
#7456=ORIENTED_EDGE ( 'NONE', *, *, #5447, .F. ) ;
#7459=ORIENTED_EDGE ( 'NONE', *, *, #7700, .T. ) ;
#7468=EDGE_LOOP ( 'NONE', ( #8269, #5582 ) ) ;
#7479=VERTEX_POINT ( 'NONE', #5618 ) ;
#7499=VECTOR ( 'NONE', #1531, 1000.000000000000000 ) ;
#7511=ORIENTED_EDGE ( 'NONE', *, *, #3692, .F. ) ;
#7512=DIRECTION ( 'NONE',  ( 1.154721252774410375E-34, -3.250006781153453386E-32, 1.000000000000000000 ) ) ;
#7538=LINE ( 'NONE', #9327, #502 ) ;
#7578=CARTESIAN_POINT ( 'NONE',  ( 11.00000000000003730, -19.99999999999999645, 9.850000000000040501 ) ) ;
#7613=LINE ( 'NONE', #1558, #8689 ) ;
#7619=AXIS2_PLACEMENT_3D ( 'NONE', #9421, #9488, #5454 ) ;
#7620=EDGE_CURVE ( 'NONE', #9518, #9949, #1937, .T. ) ;
#7622=PRODUCT_DEFINITION_SHAPE ( 'NONE', 'NONE',  #6898 ) ;
#7656=VECTOR ( 'NONE', #1294, 1000.000000000000000 ) ;
#7694=FACE_OUTER_BOUND ( 'NONE', #10865, .T. ) ;
#7700=EDGE_CURVE ( 'NONE', #3671, #5846, #912, .T. ) ;
#7738=ORIENTED_EDGE ( 'NONE', *, *, #4984, .T. ) ;
#7744=CARTESIAN_POINT ( 'NONE',  ( 15.00000000000003375, 30.00000000000001776, -6.000000000000013323 ) ) ;
#7760=ORIENTED_EDGE ( 'NONE', *, *, #2247, .F. ) ;
#7778=DIRECTION ( 'NONE',  ( 1.000000000000000000, 1.849040895279789448E-31, -6.938893903907224680E-17 ) ) ;
#7779=ADVANCED_FACE ( 'NONE', ( #11933 ), #10102, .F. ) ;
#7785=ORIENTED_EDGE ( 'NONE', *, *, #10041, .F. ) ;
#7834=ORIENTED_EDGE ( 'NONE', *, *, #306, .T. ) ;
#7851=ADVANCED_FACE ( 'NONE', ( #4321 ), #12191, .F. ) ;
#7885=ORIENTED_EDGE ( 'NONE', *, *, #527, .F. ) ;
#7898=EDGE_CURVE ( 'NONE', #5309, #4808, #11443, .T. ) ;
#7905=AXIS2_PLACEMENT_3D ( 'NONE', #9142, #328, #10949 ) ;
#7906=AXIS2_PLACEMENT_3D ( 'NONE', #1852, #9687, #881 ) ;
#7954=EDGE_CURVE ( 'NONE', #5440, #11959, #7538, .T. ) ;
#7965=DIRECTION ( 'NONE',  ( 0.000000000000000000, 0.000000000000000000, -1.000000000000000000 ) ) ;
#7966=ORIENTED_EDGE ( 'NONE', *, *, #12552, .T. ) ;
#7972=DIRECTION ( 'NONE',  ( 0.000000000000000000, 0.000000000000000000, 1.000000000000000000 ) ) ;
#7990=VERTEX_POINT ( 'NONE', #705 ) ;
#8005=ORIENTED_EDGE ( 'NONE', *, *, #5620, .F. ) ;
#8050=FACE_OUTER_BOUND ( 'NONE', #2390, .T. ) ;
#8137=AXIS2_PLACEMENT_3D ( 'NONE', #2315, #3232, #7965 ) ;
#8170=VECTOR ( 'NONE', #9465, 1000.000000000000000 ) ;
#8180=PLANE ( 'NONE',  #3512 ) ;
#8236=VECTOR ( 'NONE', #8300, 1000.000000000000000 ) ;
#8237=AXIS2_PLACEMENT_3D ( 'NONE', #4491, #7512, #11448 ) ;
#8239=CARTESIAN_POINT ( 'NONE',  ( 11.00000000000001599, -12.50000000000000178, 5.000000000000007994 ) ) ;
#8240=ORIENTED_EDGE ( 'NONE', *, *, #5572, .F. ) ;
#8246=EDGE_CURVE ( 'NONE', #8622, #837, #10158, .T. ) ;
#8247=FACE_OUTER_BOUND ( 'NONE', #1604, .T. ) ;
#8256=CARTESIAN_POINT ( 'NONE',  ( 11.00000000000002665, 12.50000000000000000, 5.000000000000004441 ) ) ;
#8267=DIRECTION ( 'NONE',  ( 0.000000000000000000, 4.478906847412192569E-32, -1.000000000000000000 ) ) ;
#8269=ORIENTED_EDGE ( 'NONE', *, *, #4784, .F. ) ;
#8300=DIRECTION ( 'NONE',  ( -1.848892746611746419E-31, -1.000000000000000000, 3.250006781153460502E-32 ) ) ;
#8304=CARTESIAN_POINT ( 'NONE',  ( 11.00000000000003020, -30.00000000000000000, 25.00000000000007105 ) ) ;
#8316=DIRECTION ( 'NONE',  ( -1.848892746611746419E-31, -1.000000000000000000, 3.250006781153460502E-32 ) ) ;
#8331=DIRECTION ( 'NONE',  ( 1.154721252774410375E-34, 3.250006781153453386E-32, -1.000000000000000000 ) ) ;
#8342=ORIENTED_EDGE ( 'NONE', *, *, #11702, .F. ) ;
#8387=LINE ( 'NONE', #534, #8170 ) ;
#8392=DIRECTION ( 'NONE',  ( -1.848892746611746419E-31, -1.000000000000000000, -3.250006781153453386E-32 ) ) ;
#8405=EDGE_CURVE ( 'NONE', #1045, #499, #5530, .T. ) ;
#8410=DIRECTION ( 'NONE',  ( 6.938893903907224680E-17, -3.250006781153453386E-32, 1.000000000000000000 ) ) ;
#8413=DIRECTION ( 'NONE',  ( 0.000000000000000000, 0.000000000000000000, -1.000000000000000000 ) ) ;
#8467=DIRECTION ( 'NONE',  ( -1.000000000000000000, -1.848892746611742259E-31, 1.154721252774410589E-34 ) ) ;
#8472=ORIENTED_EDGE ( 'NONE', *, *, #11707, .T. ) ;
#8552=ORIENTED_EDGE ( 'NONE', *, *, #4760, .T. ) ;
#8563=ADVANCED_FACE ( 'NONE', ( #6012 ), #153, .F. ) ;
#8608=FACE_OUTER_BOUND ( 'NONE', #6554, .T. ) ;
#8613=VERTEX_POINT ( 'NONE', #4018 ) ;
#8620=AXIS2_PLACEMENT_3D ( 'NONE', #3277, #7190, #2300 ) ;
#8622=VERTEX_POINT ( 'NONE', #9157 ) ;
#8624=CARTESIAN_POINT ( 'NONE',  ( 11.00000000000003020, 30.00000000000000000, -9.742497179615118866E-31 ) ) ;
#8627=AXIS2_PLACEMENT_3D ( 'NONE', #11112, #3022, #5064 ) ;
#8659=CARTESIAN_POINT ( 'NONE',  ( 9.000000000000017764, -12.50000000000000000, 5.000000000000007994 ) ) ;
#8661=DIRECTION ( 'NONE',  ( -1.848892746611746419E-31, -1.000000000000000000, 3.250006781153460502E-32 ) ) ;
#8670=ORIENTED_EDGE ( 'NONE', *, *, #3692, .T. ) ;
#8671=EDGE_CURVE ( 'NONE', #10853, #7453, #2418, .T. ) ;
#8677=AXIS2_PLACEMENT_3D ( 'NONE', #1614, #5735, #11481 ) ;
#8678=ORIENTED_EDGE ( 'NONE', *, *, #5447, .T. ) ;
#8689=VECTOR ( 'NONE', #5493, 1000.000000000000000 ) ;
#8711=EDGE_CURVE ( 'NONE', #5309, #10795, #2353, .T. ) ;
#8735=( LENGTH_UNIT ( ) NAMED_UNIT ( * ) SI_UNIT ( .MILLI., .METRE. ) );
#8759=ORIENTED_EDGE ( 'NONE', *, *, #12744, .T. ) ;
#8774=AXIS2_PLACEMENT_3D ( 'NONE', #1889, #10642, #5817 ) ;
#8783=DIRECTION ( 'NONE',  ( 1.000000000000000000, 1.849040895279789448E-31, -6.938893903907224680E-17 ) ) ;
#8791=EDGE_LOOP ( 'NONE', ( #9764, #5473, #1906, #1898 ) ) ;
#8864=VERTEX_POINT ( 'NONE', #4659 ) ;
#8872=ORIENTED_EDGE ( 'NONE', *, *, #11724, .F. ) ;
#8881=ORIENTED_EDGE ( 'NONE', *, *, #7620, .F. ) ;
#8883=DIRECTION ( 'NONE',  ( 0.000000000000000000, 0.000000000000000000, 1.000000000000000000 ) ) ;
#8892=VECTOR ( 'NONE', #1918, 1000.000000000000000 ) ;
#8931=CARTESIAN_POINT ( 'NONE',  ( 11.00000000000003375, 12.50000000000000000, -4.062508476441825628E-31 ) ) ;
#8944=VERTEX_POINT ( 'NONE', #5931 ) ;
#8957=FACE_OUTER_BOUND ( 'NONE', #8791, .T. ) ;
#9008=CARTESIAN_POINT ( 'NONE',  ( 11.00000000000003020, 30.00000000000000000, -9.742497179615118866E-31 ) ) ;
#9009=DIRECTION ( 'NONE',  ( 0.000000000000000000, 0.000000000000000000, 1.000000000000000000 ) ) ;
#9039=SHAPE_DEFINITION_REPRESENTATION ( #7622, #71 ) ;
#9040=COLOUR_RGB ( '', 0.09019608, 0.27058824, 0.51372549) ;
#9075=EDGE_CURVE ( 'NONE', #4417, #7479, #3941, .T. ) ;
#9098=EDGE_CURVE ( 'NONE', #7479, #1463, #10251, .T. ) ;
#9117=ORIENTED_EDGE ( 'NONE', *, *, #10876, .T. ) ;
#9142=CARTESIAN_POINT ( 'NONE',  ( 9.000000000000031974, -6.123233995736753463E-16, 20.00000000000003553 ) ) ;
#9145=DIRECTION ( 'NONE',  ( 1.000000000000000000, 1.849040895279789448E-31, -6.938893903907224680E-17 ) ) ;
#9149=LINE ( 'NONE', #2279, #4148 ) ;
#9157=CARTESIAN_POINT ( 'NONE',  ( 12.94787914004602847, -12.49999999999999645, 5.638155724715463002 ) ) ;
#9188=ORIENTED_EDGE ( 'NONE', *, *, #9075, .T. ) ;
#9253=AXIS2_PLACEMENT_3D ( 'NONE', #1093, #9836, #8883 ) ;
#9255=CARTESIAN_POINT ( 'NONE',  ( 11.00000000000001599, 19.99999999999999645, 12.00000000000003020 ) ) ;
#9276=ORIENTED_EDGE ( 'NONE', *, *, #8246, .T. ) ;
#9288=ORIENTED_EDGE ( 'NONE', *, *, #4049, .F. ) ;
#9318=EDGE_CURVE ( 'NONE', #10196, #8613, #6517, .T. ) ;
#9327=CARTESIAN_POINT ( 'NONE',  ( 21.00000000000003197, 30.00000000000000000, 5.000000000000004441 ) ) ;
#9361=FACE_BOUND ( 'NONE', #1549, .T. ) ;
#9413=DIRECTION ( 'NONE',  ( 0.000000000000000000, 0.000000000000000000, -1.000000000000000000 ) ) ;
#9414=ORIENTED_EDGE ( 'NONE', *, *, #11800, .F. ) ;
#9419=ORIENTED_EDGE ( 'NONE', *, *, #576, .T. ) ;
#9421=CARTESIAN_POINT ( 'NONE',  ( 9.000000000000028422, 30.00000000000000000, 1.387778780781438526E-16 ) ) ;
#9433=CARTESIAN_POINT ( 'NONE',  ( 9.000000000000028422, -30.00000000000000000, 5.000000000000011546 ) ) ;
#9434=CARTESIAN_POINT ( 'NONE',  ( 21.00000000000004974, -12.49999999999999289, 5.000000000000007994 ) ) ;
#9442=ORIENTED_EDGE ( 'NONE', *, *, #11707, .F. ) ;
#9448=MECHANICAL_DESIGN_GEOMETRIC_PRESENTATION_REPRESENTATION('',(#12153),#11111);
#9465=DIRECTION ( 'NONE',  ( -1.848892746611746419E-31, -1.000000000000000000, 3.250006781153460502E-32 ) ) ;
#9488=DIRECTION ( 'NONE',  ( 1.000000000000000000, 1.849040895279789667E-31, -6.938893903907224680E-17 ) ) ;
#9517=DIRECTION ( 'NONE',  ( -1.848892746611746419E-31, -1.000000000000000000, 3.250006781153460502E-32 ) ) ;
#9518=VERTEX_POINT ( 'NONE', #8239 ) ;
#9538=VECTOR ( 'NONE', #7778, 1000.000000000000000 ) ;
#9548=( NAMED_UNIT ( * ) SI_UNIT ( $, .STERADIAN. ) SOLID_ANGLE_UNIT ( ) );
#9617=ADVANCED_FACE ( 'NONE', ( #2389 ), #5339, .F. ) ;
#9618=ORIENTED_EDGE ( 'NONE', *, *, #4984, .F. ) ;
#9620=CARTESIAN_POINT ( 'NONE',  ( 11.00000000000001599, -12.49999999999999645, -4.423544863740860615E-14 ) ) ;
#9624=CIRCLE ( 'NONE', #11910, 2.149999999999994138 ) ;
#9650=EDGE_CURVE ( 'NONE', #5440, #937, #508, .T. ) ;
#9673=SURFACE_STYLE_FILL_AREA ( #2890 ) ;
#9682=AXIS2_PLACEMENT_3D ( 'NONE', #3182, #198, #6056 ) ;
#9684=CYLINDRICAL_SURFACE ( 'NONE', #9706, 4.000000000000008882 ) ;
#9687=DIRECTION ( 'NONE',  ( -1.848892746611742259E-31, 1.000000000000000000, -3.250006781153460502E-32 ) ) ;
#9704=ORIENTED_EDGE ( 'NONE', *, *, #5663, .F. ) ;
#9706=AXIS2_PLACEMENT_3D ( 'NONE', #10852, #2902, #11774 ) ;
#9708=AXIS2_PLACEMENT_3D ( 'NONE', #3816, #12645, #3936 ) ;
#9710=CIRCLE ( 'NONE', #265, 6.000000000000013323 ) ;
#9732=VERTEX_POINT ( 'NONE', #12306 ) ;
#9764=ORIENTED_EDGE ( 'NONE', *, *, #6766, .F. ) ;
#9767=AXIS2_PLACEMENT_3D ( 'NONE', #11152, #3251, #6127 ) ;
#9787=CIRCLE ( 'NONE', #8774, 2.149999999999999023 ) ;
#9793=DIRECTION ( 'NONE',  ( 1.000000000000000000, 1.849040895279789448E-31, -6.938893903907224680E-17 ) ) ;
#9816=ORIENTED_EDGE ( 'NONE', *, *, #6646, .T. ) ;
#9830=EDGE_CURVE ( 'NONE', #12174, #8613, #361, .T. ) ;
#9836=DIRECTION ( 'NONE',  ( 1.848892746611746419E-31, 1.000000000000000000, -3.250006781153460502E-32 ) ) ;
#9870=COLOUR_RGB ( '', 0.09019608, 0.27058824, 0.51372549) ;
#9885=ORIENTED_EDGE ( 'NONE', *, *, #772, .F. ) ;
#9919=MANIFOLD_SOLID_BREP ( 'Move Face1', #2746 ) ;
#9928=VECTOR ( 'NONE', #6730, 1000.000000000000000 ) ;
#9949=VERTEX_POINT ( 'NONE', #6679 ) ;
#9968=CARTESIAN_POINT ( 'NONE',  ( 15.00000000000003375, -12.49999999999999645, 3.994800001834461867E-31 ) ) ;
#9983=ORIENTED_EDGE ( 'NONE', *, *, #6786, .T. ) ;
#9988=VECTOR ( 'NONE', #3465, 1000.000000000000000 ) ;
#9992=ORIENTED_EDGE ( 'NONE', *, *, #576, .F. ) ;
#10031=FACE_BOUND ( 'NONE', #7468, .T. ) ;
#10041=EDGE_CURVE ( 'NONE', #2489, #11959, #3072, .T. ) ;
#10064=AXIS2_PLACEMENT_3D ( 'NONE', #6016, #3076, #4214 ) ;
#10101=APPLICATION_CONTEXT ( 'automotive_design' ) ;
#10102=PLANE ( 'NONE',  #9767 ) ;
#10119=DIRECTION ( 'NONE',  ( -6.938893903907224680E-17, 1.040834085586079721E-15, -1.000000000000000000 ) ) ;
#10138=ORIENTED_EDGE ( 'NONE', *, *, #9098, .T. ) ;
#10158=CIRCLE ( 'NONE', #6060, 6.000000000000013323 ) ;
#10196=VERTEX_POINT ( 'NONE', #6401 ) ;
#10200=VECTOR ( 'NONE', #5177, 1000.000000000000000 ) ;
#10209=CYLINDRICAL_SURFACE ( 'NONE', #10782, 2.149999999999999023 ) ;
#10214=ORIENTED_EDGE ( 'NONE', *, *, #9075, .F. ) ;
#10235=CARTESIAN_POINT ( 'NONE',  ( 9.000000000000017764, -12.49999999999999645, -1.576761677324507637E-16 ) ) ;
#10240=CIRCLE ( 'NONE', #10064, 2.149999999999994138 ) ;
#10251=CIRCLE ( 'NONE', #4091, 2.149999999999994138 ) ;
#10252=FACE_OUTER_BOUND ( 'NONE', #902, .T. ) ;
#10259=AXIS2_PLACEMENT_3D ( 'NONE', #2791, #7066, #6644 ) ;
#10279=( GEOMETRIC_REPRESENTATION_CONTEXT ( 3 ) GLOBAL_UNCERTAINTY_ASSIGNED_CONTEXT ( ( #1818 ) ) GLOBAL_UNIT_ASSIGNED_CONTEXT ( ( #8735, #1233, #2896 ) ) REPRESENTATION_CONTEXT ( 'NONE', 'WORKASPACE' ) );
#10285=ORIENTED_EDGE ( 'NONE', *, *, #5572, .T. ) ;
#10308=CARTESIAN_POINT ( 'NONE',  ( 11.00000000000003375, -3.490243377569932395E-16, 22.15000000000003411 ) ) ;
#10309=VECTOR ( 'NONE', #6713, 1000.000000000000000 ) ;
#10330=CIRCLE ( 'NONE', #4794, 6.000000000000013323 ) ;
#10366=ADVANCED_FACE ( 'NONE', ( #8050 ), #1943, .T. ) ;
#10391=ORIENTED_EDGE ( 'NONE', *, *, #4980, .T. ) ;
#10407=ORIENTED_EDGE ( 'NONE', *, *, #12538, .T. ) ;
#10411=CARTESIAN_POINT ( 'NONE',  ( 15.00000000000003375, 30.00000000000001776, 4.000000000000008882 ) ) ;
#10448=UNCERTAINTY_MEASURE_WITH_UNIT (LENGTH_MEASURE( 1.000000000000000082E-05 ), #6131, 'distance_accuracy_value', 'NONE');
#10454=CARTESIAN_POINT ( 'NONE',  ( 9.000000000000017764, 19.99999999999999645, 9.850000000000029843 ) ) ;
#10466=ORIENTED_EDGE ( 'NONE', *, *, #6576, .T. ) ;
#10500=CARTESIAN_POINT ( 'NONE',  ( 11.00000000000001599, 19.99999999999999645, 9.850000000000029843 ) ) ;
#10511=DIRECTION ( 'NONE',  ( 0.000000000000000000, 0.000000000000000000, 1.000000000000000000 ) ) ;
#10521=CARTESIAN_POINT ( 'NONE',  ( 15.00000000000003375, 30.00000000000001776, -9.742497179615118866E-31 ) ) ;
#10585=CARTESIAN_POINT ( 'NONE',  ( 11.00000000000003375, -19.99999999999999645, 12.00000000000003553 ) ) ;
#10616=VECTOR ( 'NONE', #737, 1000.000000000000000 ) ;
#10642=DIRECTION ( 'NONE',  ( 1.000000000000000000, 1.849040895279789448E-31, -6.938893903907224680E-17 ) ) ;
#10646=VERTEX_POINT ( 'NONE', #2663 ) ;
#10661=PLANE ( 'NONE',  #7906 ) ;
#10711=( LENGTH_UNIT ( ) NAMED_UNIT ( * ) SI_UNIT ( .MILLI., .METRE. ) );
#10712=ORIENTED_EDGE ( 'NONE', *, *, #3431, .F. ) ;
#10727=ORIENTED_EDGE ( 'NONE', *, *, #8246, .F. ) ;
#10751=EDGE_CURVE ( 'NONE', #3763, #11641, #6589, .T. ) ;
#10759=DIRECTION ( 'NONE',  ( 1.000000000000000000, 1.849040895279789448E-31, -6.938893903907224680E-17 ) ) ;
#10762=APPLICATION_CONTEXT ( 'automotive_design' ) ;
#10782=AXIS2_PLACEMENT_3D ( 'NONE', #2321, #3482, #5992 ) ;
#10795=VERTEX_POINT ( 'NONE', #5985 ) ;
#10829=CARTESIAN_POINT ( 'NONE',  ( 11.00000000000003375, -6.123233995736744589E-16, 17.85000000000003695 ) ) ;
#10852=CARTESIAN_POINT ( 'NONE',  ( 15.00000000000003375, 30.00000000000001776, -9.742497179615118866E-31 ) ) ;
#10853=VERTEX_POINT ( 'NONE', #3304 ) ;
#10855=DIRECTION ( 'NONE',  ( 1.000000000000000000, 1.849040895279789448E-31, -6.938893903907224680E-17 ) ) ;
#10865=EDGE_LOOP ( 'NONE', ( #12544, #12612, #10407, #9276 ) ) ;
#10876=EDGE_CURVE ( 'NONE', #9949, #12174, #3176, .T. ) ;
#10885=CARTESIAN_POINT ( 'NONE',  ( 11.00000000000003020, 30.00000000000000000, 4.999999999999999112 ) ) ;
#10888=VECTOR ( 'NONE', #9517, 1000.000000000000000 ) ;
#10904=CARTESIAN_POINT ( 'NONE',  ( 9.000000000000031974, 12.50000000000000000, 5.000000000000004441 ) ) ;
#10912=ADVANCED_FACE ( 'NONE', ( #9361, #6491, #12115, #2196 ), #619, .F. ) ;
#10942=CARTESIAN_POINT ( 'NONE',  ( 12.94787914004603557, 12.50000000000000000, 5.638155724715463002 ) ) ;
#10943=ADVANCED_FACE ( 'NONE', ( #12420 ), #3595, .T. ) ;
#10949=DIRECTION ( 'NONE',  ( 0.000000000000000000, 4.478906847412178337E-32, -1.000000000000000000 ) ) ;
#10954=CARTESIAN_POINT ( 'NONE',  ( 11.00000000000001599, 19.99999999999999645, 12.00000000000003020 ) ) ;
#11038=DIRECTION ( 'NONE',  ( 1.848892746611746419E-31, 1.000000000000000000, -3.250006781153460502E-32 ) ) ;
#11084=DIRECTION ( 'NONE',  ( 1.848892746611746419E-31, 1.000000000000000000, 3.250006781153453386E-32 ) ) ;
#11111=( GEOMETRIC_REPRESENTATION_CONTEXT ( 3 ) GLOBAL_UNCERTAINTY_ASSIGNED_CONTEXT ( ( #786 ) ) GLOBAL_UNIT_ASSIGNED_CONTEXT ( ( #10711, #6618, #9548 ) ) REPRESENTATION_CONTEXT ( 'NONE', 'WORKASPACE' ) );
#11112=CARTESIAN_POINT ( 'NONE',  ( 15.00000000000003375, 30.00000000000001776, -9.742497179615118866E-31 ) ) ;
#11138=EDGE_CURVE ( 'NONE', #1463, #7479, #10240, .T. ) ;
#11149=CARTESIAN_POINT ( 'NONE',  ( 15.00000000000003375, -12.49999999999999645, 3.994800001834461867E-31 ) ) ;
#11152=CARTESIAN_POINT ( 'NONE',  ( 21.00000000000004974, -12.49999999999999289, 5.000000000000007994 ) ) ;
#11172=PLANE ( 'NONE',  #845 ) ;
#11239=ORIENTED_EDGE ( 'NONE', *, *, #11924, .F. ) ;
#11243=EDGE_CURVE ( 'NONE', #10795, #7388, #3541, .T. ) ;
#11245=FACE_OUTER_BOUND ( 'NONE', #2876, .T. ) ;
#11254=ORIENTED_EDGE ( 'NONE', *, *, #2247, .T. ) ;
#11261=ADVANCED_BREP_SHAPE_REPRESENTATION ( '', ( #9919, #12422 ), #3113 ) ;
#11277=DIRECTION ( 'NONE',  ( 1.000000000000000000, 1.849040895279789448E-31, -6.938893903907224680E-17 ) ) ;
#11283=LINE ( 'NONE', #2468, #7656 ) ;
#11287=CARTESIAN_POINT ( 'NONE',  ( 15.00000000000003375, -12.49999999999999645, -4.000000000000000000 ) ) ;
#11307=CARTESIAN_POINT ( 'NONE',  ( 11.00000000000001599, 19.99999999999999645, 9.850000000000035172 ) ) ;
#11332=CARTESIAN_POINT ( 'NONE',  ( 11.00000000000003375, -19.99999999999999645, 9.850000000000035172 ) ) ;
#11352=ADVANCED_FACE ( 'NONE', ( #347 ), #11172, .F. ) ;
#11409=VECTOR ( 'NONE', #10119, 1000.000000000000000 ) ;
#11443=CIRCLE ( 'NONE', #7905, 2.149999999999999023 ) ;
#11448=DIRECTION ( 'NONE',  ( 1.000000000000000000, 1.848892746611742259E-31, -1.154721252774410375E-34 ) ) ;
#11453=LINE ( 'NONE', #6556, #124 ) ;
#11474=AXIS2_PLACEMENT_3D ( 'NONE', #12252, #11277, #12313 ) ;
#11481=DIRECTION ( 'NONE',  ( 0.000000000000000000, 0.000000000000000000, -1.000000000000000000 ) ) ;
#11487=EDGE_CURVE ( 'NONE', #8864, #499, #7239, .T. ) ;
#11504=ORIENTED_EDGE ( 'NONE', *, *, #9650, .T. ) ;
#11560=ADVANCED_FACE ( 'NONE', ( #8957 ), #11876, .F. ) ;
#11569=CARTESIAN_POINT ( 'NONE',  ( 9.000000000000031974, -6.123233995736752477E-16, 17.85000000000003695 ) ) ;
#11641=VERTEX_POINT ( 'NONE', #1232 ) ;
#11650=ORIENTED_EDGE ( 'NONE', *, *, #12744, .F. ) ;
#11702=EDGE_CURVE ( 'NONE', #349, #9732, #2522, .T. ) ;
#11706=EDGE_CURVE ( 'NONE', #8622, #8864, #9149, .T. ) ;
#11707=EDGE_CURVE ( 'NONE', #937, #2489, #1552, .T. ) ;
#11712=EDGE_LOOP ( 'NONE', ( #1026, #5000, #7399, #10712, #10285, #7138, #11239, #7785 ) ) ;
#11724=EDGE_CURVE ( 'NONE', #9949, #4174, #11283, .T. ) ;
#11738=LINE ( 'NONE', #7744, #3044 ) ;
#11745=DIRECTION ( 'NONE',  ( 1.000000000000000000, 1.848892746611742259E-31, -1.154721252774410375E-34 ) ) ;
#11753=CARTESIAN_POINT ( 'NONE',  ( 11.00000000000001599, 19.99999999999999645, 12.00000000000003020 ) ) ;
#11756=DIRECTION ( 'NONE',  ( 1.000000000000000000, 1.849040895279789448E-31, -6.938893903907224680E-17 ) ) ;
#11774=DIRECTION ( 'NONE',  ( 0.000000000000000000, 0.000000000000000000, -1.000000000000000000 ) ) ;
#11800=EDGE_CURVE ( 'NONE', #3356, #5846, #1808, .T. ) ;
#11820=EDGE_CURVE ( 'NONE', #8944, #1393, #3753, .T. ) ;
#11833=DIRECTION ( 'NONE',  ( -1.848892746611746419E-31, -1.000000000000000000, 3.250006781153460502E-32 ) ) ;
#11834=ORIENTED_EDGE ( 'NONE', *, *, #527, .T. ) ;
#11836=DIRECTION ( 'NONE',  ( 6.938893903907224680E-17, -1.040834085586079721E-15, 1.000000000000000000 ) ) ;
#11876=CYLINDRICAL_SURFACE ( 'NONE', #3551, 2.149999999999999023 ) ;
#11907=LINE ( 'NONE', #4236, #7335 ) ;
#11910=AXIS2_PLACEMENT_3D ( 'NONE', #11753, #9793, #1109 ) ;
#11924=EDGE_CURVE ( 'NONE', #11959, #10196, #6652, .T. ) ;
#11932=CARTESIAN_POINT ( 'NONE',  ( 9.000000000000031974, -3.490243377569940777E-16, 22.15000000000003055 ) ) ;
#11933=FACE_OUTER_BOUND ( 'NONE', #12114, .T. ) ;
#11950=CARTESIAN_POINT ( 'NONE',  ( 9.000000000000035527, -19.99999999999999645, 12.00000000000003553 ) ) ;
#11959=VERTEX_POINT ( 'NONE', #12704 ) ;
#11974=VERTEX_POINT ( 'NONE', #10942 ) ;
#11978=DIRECTION ( 'NONE',  ( -6.938893903907224680E-17, 3.250006781153453386E-32, -1.000000000000000000 ) ) ;
#11979=ORIENTED_EDGE ( 'NONE', *, *, #10041, .T. ) ;
#11992=DIRECTION ( 'NONE',  ( 0.000000000000000000, 0.000000000000000000, 1.000000000000000000 ) ) ;
#12064=( NAMED_UNIT ( * ) SI_UNIT ( $, .STERADIAN. ) SOLID_ANGLE_UNIT ( ) );
#12072=CARTESIAN_POINT ( 'NONE',  ( 11.00000000000003020, 30.00000000000000000, -7.347880794884148332E-16 ) ) ;
#12114=EDGE_LOOP ( 'NONE', ( #604, #6079, #3193, #298 ) ) ;
#12115=FACE_BOUND ( 'NONE', #2466, .T. ) ;
#12145=VECTOR ( 'NONE', #11833, 1000.000000000000000 ) ;
#12149=ORIENTED_EDGE ( 'NONE', *, *, #8671, .T. ) ;
#12153=STYLED_ITEM ( 'NONE', ( #12476 ), #9919 ) ;
#12174=VERTEX_POINT ( 'NONE', #8304 ) ;
#12191=PLANE ( 'NONE',  #3196 ) ;
#12230=ORIENTED_EDGE ( 'NONE', *, *, #7898, .F. ) ;
#12232=CIRCLE ( 'NONE', #6678, 2.149999999999999023 ) ;
#12247=DIRECTION ( 'NONE',  ( 1.000000000000000000, 1.849040895279789667E-31, -6.938893903907224680E-17 ) ) ;
#12252=CARTESIAN_POINT ( 'NONE',  ( 9.000000000000017764, 19.99999999999999645, 12.00000000000003020 ) ) ;
#12274=VECTOR ( 'NONE', #11978, 1000.000000000000000 ) ;
#12282=CARTESIAN_POINT ( 'NONE',  ( 11.00000000000003375, 12.50000000000000000, 5.000000000000004441 ) ) ;
#12286=ORIENTED_EDGE ( 'NONE', *, *, #5832, .T. ) ;
#12293=ORIENTED_EDGE ( 'NONE', *, *, #7200, .T. ) ;
#12306=CARTESIAN_POINT ( 'NONE',  ( 15.00000000000003375, 12.50000000000000000, -4.000000000000000000 ) ) ;
#12311=CARTESIAN_POINT ( 'NONE',  ( 15.00000000000003375, -12.49999999999999645, -6.000000000000000000 ) ) ;
#12313=DIRECTION ( 'NONE',  ( 0.000000000000000000, 0.000000000000000000, -1.000000000000000000 ) ) ;
#12326=ORIENTED_EDGE ( 'NONE', *, *, #6020, .T. ) ;
#12329=AXIS2_PLACEMENT_3D ( 'NONE', #10521, #8661, #2821 ) ;
#12350=DIRECTION ( 'NONE',  ( -1.848892746611746419E-31, -1.000000000000000000, 3.250006781153460502E-32 ) ) ;
#12372=STYLED_ITEM ( 'NONE', ( #7041 ), #11261 ) ;
#12392=VECTOR ( 'NONE', #3751, 1000.000000000000000 ) ;
#12420=FACE_OUTER_BOUND ( 'NONE', #7070, .T. ) ;
#12422=AXIS2_PLACEMENT_3D ( 'NONE', #5707, #7392, #6428 ) ;
#12430=CARTESIAN_POINT ( 'NONE',  ( 11.00000000000001599, 19.99999999999999645, 14.15000000000002878 ) ) ;
#12476=PRESENTATION_STYLE_ASSIGNMENT (( #6739 ) ) ;
#12538=EDGE_CURVE ( 'NONE', #11974, #8622, #6889, .T. ) ;
#12540=FILL_AREA_STYLE_COLOUR ( '', #9040 ) ;
#12544=ORIENTED_EDGE ( 'NONE', *, *, #4760, .F. ) ;
#12552=EDGE_CURVE ( 'NONE', #9732, #1045, #6227, .T. ) ;
#12553=CARTESIAN_POINT ( 'NONE',  ( 15.00000000000003375, 12.50000000000000000, 6.000000000000000000 ) ) ;
#12584=FACE_OUTER_BOUND ( 'NONE', #7135, .T. ) ;
#12604=LINE ( 'NONE', #6925, #10616 ) ;
#12609=ORIENTED_EDGE ( 'NONE', *, *, #2991, .F. ) ;
#12612=ORIENTED_EDGE ( 'NONE', *, *, #854, .T. ) ;
#12619=ORIENTED_EDGE ( 'NONE', *, *, #854, .F. ) ;
#12645=DIRECTION ( 'NONE',  ( 1.154721252774410375E-34, -3.250006781153453386E-32, 1.000000000000000000 ) ) ;
#12704=CARTESIAN_POINT ( 'NONE',  ( 9.000000000000028422, 30.00000000000000000, 5.000000000000004441 ) ) ;
#12707=CIRCLE ( 'NONE', #11474, 2.149999999999999023 ) ;
#12727=ORIENTED_EDGE ( 'NONE', *, *, #11706, .T. ) ;
#12733=ORIENTED_EDGE ( 'NONE', *, *, #11820, .F. ) ;
#12744=EDGE_CURVE ( 'NONE', #7136, #8944, #9710, .T. ) ;
ENDSEC;
END-ISO-10303-21;
